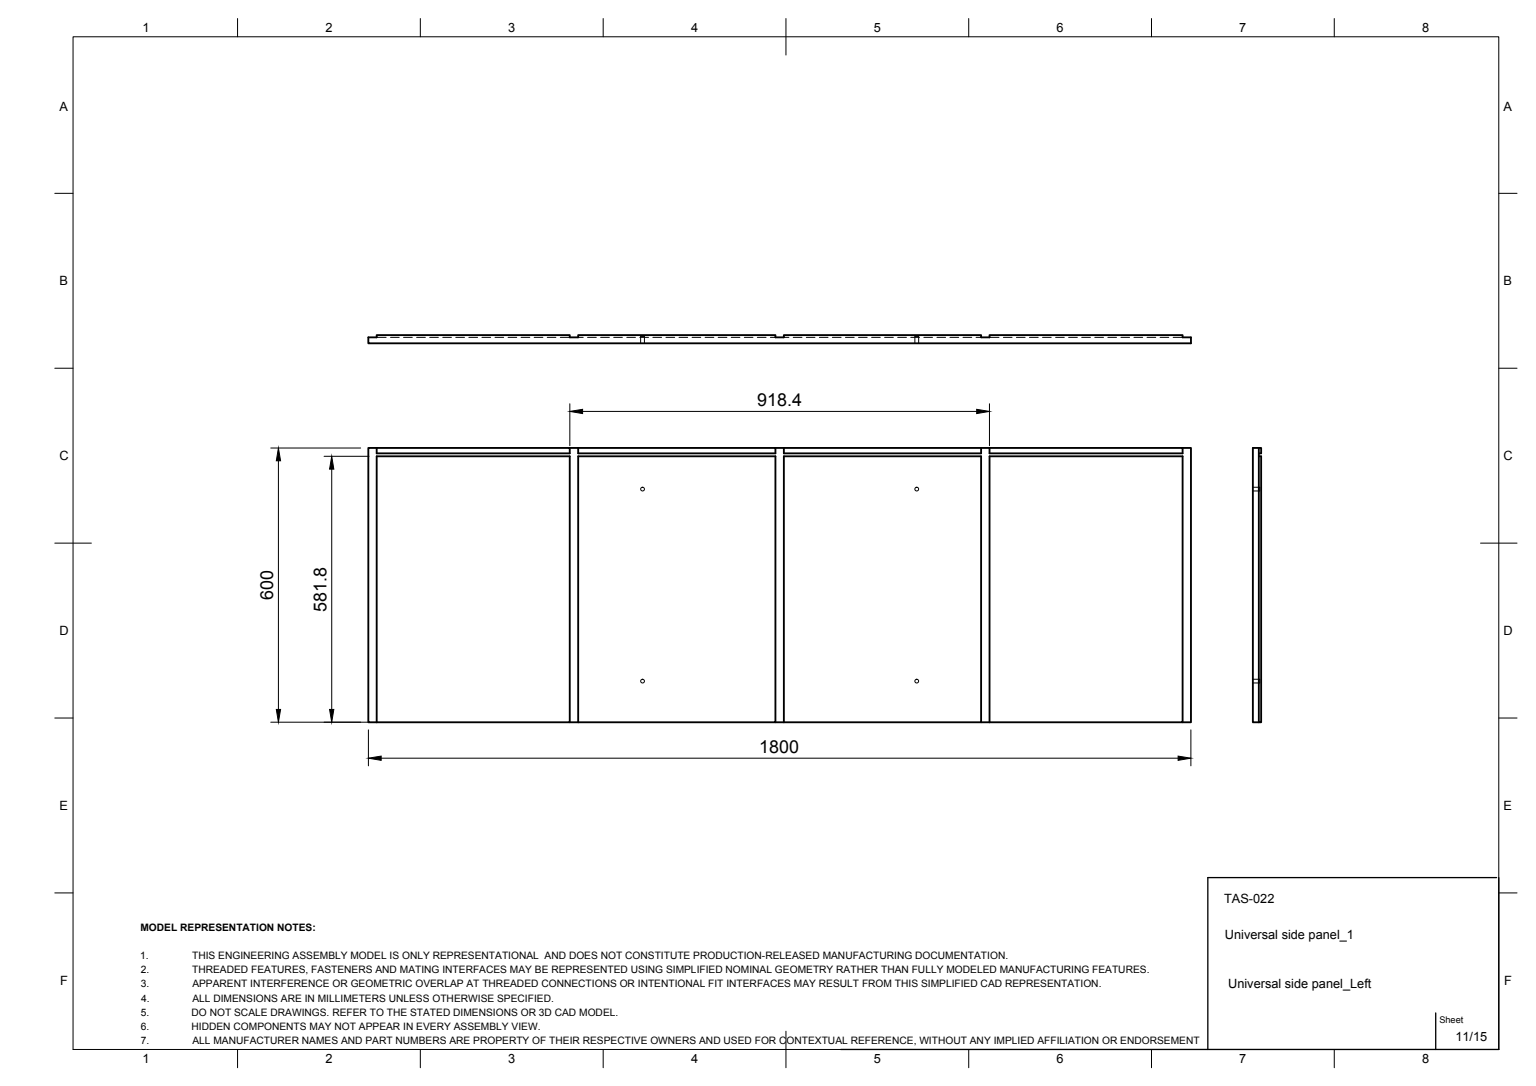
ISO-10303-21;
HEADER;
/* Generated by software containing ST-Developer
 * from STEP Tools, Inc. (www.steptools.com) 
 */

FILE_DESCRIPTION(
/* description */ (''),
/* implementation_level */ '2;1');

FILE_NAME(
/* name */ 'Universal side panel_Left.step',
/* time_stamp */ '2026-11-15T21:02:08-08:00',
/* author */ (''),
/* organization */ (''),
/* preprocessor_version */ 'ST-DEVELOPER v20.2',
/* originating_system */ 'Autodesk Translation Framework v15.17.0.0',
/* authorisation */ '');

FILE_SCHEMA (('AUTOMOTIVE_DESIGN { 1 0 10303 214 3 1 1 }'));
ENDSEC;

DATA;
#10=MECHANICAL_DESIGN_GEOMETRIC_PRESENTATION_REPRESENTATION('',(#613),#31566);
#413=FACE_BOUND('',#1182,.T.);
#414=FACE_BOUND('',#1183,.T.);
#415=FACE_BOUND('',#1184,.T.);
#416=FACE_BOUND('',#1185,.T.);
#480=CIRCLE('',#6173,0.409999999999997);
#481=CIRCLE('',#6174,0.409999999999997);
#482=CIRCLE('',#6177,0.409999999999997);
#483=CIRCLE('',#6178,0.409999999999997);
#484=CIRCLE('',#6181,0.409999999999997);
#485=CIRCLE('',#6182,0.409999999999997);
#486=CIRCLE('',#6185,0.409999999999997);
#487=CIRCLE('',#6186,0.409999999999997);
#567=CYLINDRICAL_SURFACE('',#6172,0.409999999999997);
#568=CYLINDRICAL_SURFACE('',#6176,0.409999999999997);
#569=CYLINDRICAL_SURFACE('',#6180,0.409999999999997);
#570=CYLINDRICAL_SURFACE('',#6184,0.409999999999997);
#583=SHAPE_REPRESENTATION_RELATIONSHIP('SRR','None',#31647,#598);
#598=ADVANCED_BREP_SHAPE_REPRESENTATION('',(#628),#31562);
#613=STYLED_ITEM('',(#31723),#628);
#628=MANIFOLD_SOLID_BREP('Body1',#5726);
#836=FACE_OUTER_BOUND('',#1137,.T.);
#837=FACE_OUTER_BOUND('',#1138,.T.);
#838=FACE_OUTER_BOUND('',#1139,.T.);
#839=FACE_OUTER_BOUND('',#1140,.T.);
#840=FACE_OUTER_BOUND('',#1141,.T.);
#841=FACE_OUTER_BOUND('',#1142,.T.);
#842=FACE_OUTER_BOUND('',#1143,.T.);
#843=FACE_OUTER_BOUND('',#1144,.T.);
#844=FACE_OUTER_BOUND('',#1145,.T.);
#845=FACE_OUTER_BOUND('',#1146,.T.);
#846=FACE_OUTER_BOUND('',#1147,.T.);
#847=FACE_OUTER_BOUND('',#1148,.T.);
#848=FACE_OUTER_BOUND('',#1149,.T.);
#849=FACE_OUTER_BOUND('',#1150,.T.);
#850=FACE_OUTER_BOUND('',#1151,.T.);
#851=FACE_OUTER_BOUND('',#1152,.T.);
#852=FACE_OUTER_BOUND('',#1153,.T.);
#853=FACE_OUTER_BOUND('',#1154,.T.);
#854=FACE_OUTER_BOUND('',#1155,.T.);
#855=FACE_OUTER_BOUND('',#1156,.T.);
#856=FACE_OUTER_BOUND('',#1157,.T.);
#857=FACE_OUTER_BOUND('',#1158,.T.);
#858=FACE_OUTER_BOUND('',#1159,.T.);
#859=FACE_OUTER_BOUND('',#1160,.T.);
#860=FACE_OUTER_BOUND('',#1161,.T.);
#861=FACE_OUTER_BOUND('',#1162,.T.);
#862=FACE_OUTER_BOUND('',#1163,.T.);
#863=FACE_OUTER_BOUND('',#1164,.T.);
#864=FACE_OUTER_BOUND('',#1165,.T.);
#865=FACE_OUTER_BOUND('',#1166,.T.);
#866=FACE_OUTER_BOUND('',#1167,.T.);
#867=FACE_OUTER_BOUND('',#1168,.T.);
#868=FACE_OUTER_BOUND('',#1169,.T.);
#869=FACE_OUTER_BOUND('',#1170,.T.);
#870=FACE_OUTER_BOUND('',#1171,.T.);
#871=FACE_OUTER_BOUND('',#1172,.T.);
#872=FACE_OUTER_BOUND('',#1173,.T.);
#873=FACE_OUTER_BOUND('',#1174,.T.);
#874=FACE_OUTER_BOUND('',#1175,.T.);
#875=FACE_OUTER_BOUND('',#1176,.T.);
#876=FACE_OUTER_BOUND('',#1177,.T.);
#877=FACE_OUTER_BOUND('',#1178,.T.);
#878=FACE_OUTER_BOUND('',#1179,.T.);
#879=FACE_OUTER_BOUND('',#1180,.T.);
#880=FACE_OUTER_BOUND('',#1181,.T.);
#881=FACE_OUTER_BOUND('',#1186,.T.);
#1137=EDGE_LOOP('',(#4945,#4946,#4947,#4948));
#1138=EDGE_LOOP('',(#4949));
#1139=EDGE_LOOP('',(#4950,#4951,#4952,#4953));
#1140=EDGE_LOOP('',(#4954));
#1141=EDGE_LOOP('',(#4955,#4956,#4957,#4958));
#1142=EDGE_LOOP('',(#4959));
#1143=EDGE_LOOP('',(#4960,#4961,#4962,#4963));
#1144=EDGE_LOOP('',(#4964));
#1145=EDGE_LOOP('',(#4965,#4966,#4967,#4968));
#1146=EDGE_LOOP('',(#4969,#4970,#4971,#4972));
#1147=EDGE_LOOP('',(#4973,#4974,#4975,#4976));
#1148=EDGE_LOOP('',(#4977,#4978,#4979,#4980));
#1149=EDGE_LOOP('',(#4981,#4982,#4983,#4984));
#1150=EDGE_LOOP('',(#4985,#4986,#4987,#4988));
#1151=EDGE_LOOP('',(#4989,#4990,#4991,#4992));
#1152=EDGE_LOOP('',(#4993,#4994,#4995,#4996));
#1153=EDGE_LOOP('',(#4997,#4998,#4999,#5000,#5001,#5002,#5003,#5004,#5005,
#5006,#5007,#5008,#5009,#5010,#5011,#5012,#5013,#5014,#5015,#5016,#5017,
#5018,#5019,#5020,#5021,#5022,#5023,#5024,#5025,#5026,#5027,#5028,#5029,
#5030,#5031,#5032));
#1154=EDGE_LOOP('',(#5033,#5034,#5035,#5036));
#1155=EDGE_LOOP('',(#5037,#5038,#5039,#5040));
#1156=EDGE_LOOP('',(#5041,#5042,#5043,#5044));
#1157=EDGE_LOOP('',(#5045,#5046,#5047,#5048));
#1158=EDGE_LOOP('',(#5049,#5050,#5051,#5052));
#1159=EDGE_LOOP('',(#5053,#5054,#5055,#5056));
#1160=EDGE_LOOP('',(#5057,#5058,#5059,#5060));
#1161=EDGE_LOOP('',(#5061,#5062,#5063,#5064));
#1162=EDGE_LOOP('',(#5065,#5066,#5067,#5068));
#1163=EDGE_LOOP('',(#5069,#5070,#5071,#5072));
#1164=EDGE_LOOP('',(#5073,#5074,#5075,#5076));
#1165=EDGE_LOOP('',(#5077,#5078,#5079,#5080));
#1166=EDGE_LOOP('',(#5081,#5082,#5083,#5084));
#1167=EDGE_LOOP('',(#5085,#5086,#5087,#5088));
#1168=EDGE_LOOP('',(#5089,#5090,#5091,#5092));
#1169=EDGE_LOOP('',(#5093,#5094,#5095,#5096));
#1170=EDGE_LOOP('',(#5097,#5098,#5099,#5100));
#1171=EDGE_LOOP('',(#5101,#5102,#5103,#5104));
#1172=EDGE_LOOP('',(#5105,#5106,#5107,#5108));
#1173=EDGE_LOOP('',(#5109,#5110,#5111,#5112));
#1174=EDGE_LOOP('',(#5113,#5114,#5115,#5116));
#1175=EDGE_LOOP('',(#5117,#5118,#5119,#5120));
#1176=EDGE_LOOP('',(#5121,#5122,#5123,#5124));
#1177=EDGE_LOOP('',(#5125,#5126,#5127,#5128));
#1178=EDGE_LOOP('',(#5129,#5130,#5131,#5132,#5133,#5134,#5135,#5136,#5137,
#5138,#5139,#5140,#5141,#5142,#5143,#5144,#5145,#5146,#5147,#5148));
#1179=EDGE_LOOP('',(#5149,#5150,#5151,#5152));
#1180=EDGE_LOOP('',(#5153,#5154,#5155,#5156,#5157,#5158,#5159,#5160,#5161,
#5162,#5163,#5164,#5165,#5166,#5167,#5168,#5169,#5170,#5171,#5172));
#1181=EDGE_LOOP('',(#5173,#5174,#5175,#5176));
#1182=EDGE_LOOP('',(#5177));
#1183=EDGE_LOOP('',(#5178));
#1184=EDGE_LOOP('',(#5179));
#1185=EDGE_LOOP('',(#5180));
#1186=EDGE_LOOP('',(#5181,#5182,#5183,#5184));
#1564=LINE('',#31172,#2071);
#1565=LINE('',#31179,#2072);
#1566=LINE('',#31186,#2073);
#1567=LINE('',#31193,#2074);
#1568=LINE('',#31199,#2075);
#1569=LINE('',#31201,#2076);
#1570=LINE('',#31203,#2077);
#1571=LINE('',#31204,#2078);
#1572=LINE('',#31208,#2079);
#1573=LINE('',#31210,#2080);
#1574=LINE('',#31212,#2081);
#1575=LINE('',#31213,#2082);
#1576=LINE('',#31217,#2083);
#1577=LINE('',#31219,#2084);
#1578=LINE('',#31221,#2085);
#1579=LINE('',#31222,#2086);
#1580=LINE('',#31226,#2087);
#1581=LINE('',#31228,#2088);
#1582=LINE('',#31230,#2089);
#1583=LINE('',#31231,#2090);
#1584=LINE('',#31235,#2091);
#1585=LINE('',#31237,#2092);
#1586=LINE('',#31239,#2093);
#1587=LINE('',#31240,#2094);
#1588=LINE('',#31244,#2095);
#1589=LINE('',#31246,#2096);
#1590=LINE('',#31248,#2097);
#1591=LINE('',#31249,#2098);
#1592=LINE('',#31253,#2099);
#1593=LINE('',#31255,#2100);
#1594=LINE('',#31257,#2101);
#1595=LINE('',#31258,#2102);
#1596=LINE('',#31262,#2103);
#1597=LINE('',#31264,#2104);
#1598=LINE('',#31266,#2105);
#1599=LINE('',#31267,#2106);
#1600=LINE('',#31270,#2107);
#1601=LINE('',#31272,#2108);
#1602=LINE('',#31274,#2109);
#1603=LINE('',#31276,#2110);
#1604=LINE('',#31277,#2111);
#1605=LINE('',#31279,#2112);
#1606=LINE('',#31281,#2113);
#1607=LINE('',#31282,#2114);
#1608=LINE('',#31284,#2115);
#1609=LINE('',#31286,#2116);
#1610=LINE('',#31287,#2117);
#1611=LINE('',#31289,#2118);
#1612=LINE('',#31291,#2119);
#1613=LINE('',#31292,#2120);
#1614=LINE('',#31294,#2121);
#1615=LINE('',#31296,#2122);
#1616=LINE('',#31298,#2123);
#1617=LINE('',#31300,#2124);
#1618=LINE('',#31301,#2125);
#1619=LINE('',#31303,#2126);
#1620=LINE('',#31305,#2127);
#1621=LINE('',#31306,#2128);
#1622=LINE('',#31308,#2129);
#1623=LINE('',#31310,#2130);
#1624=LINE('',#31311,#2131);
#1625=LINE('',#31313,#2132);
#1626=LINE('',#31315,#2133);
#1627=LINE('',#31316,#2134);
#1628=LINE('',#31319,#2135);
#1629=LINE('',#31320,#2136);
#1630=LINE('',#31323,#2137);
#1631=LINE('',#31324,#2138);
#1632=LINE('',#31327,#2139);
#1633=LINE('',#31328,#2140);
#1634=LINE('',#31331,#2141);
#1635=LINE('',#31332,#2142);
#1636=LINE('',#31334,#2143);
#1637=LINE('',#31336,#2144);
#1638=LINE('',#31339,#2145);
#1639=LINE('',#31340,#2146);
#1640=LINE('',#31343,#2147);
#1641=LINE('',#31344,#2148);
#1642=LINE('',#31347,#2149);
#1643=LINE('',#31348,#2150);
#1644=LINE('',#31351,#2151);
#1645=LINE('',#31352,#2152);
#1646=LINE('',#31354,#2153);
#1647=LINE('',#31356,#2154);
#1648=LINE('',#31359,#2155);
#1649=LINE('',#31360,#2156);
#1650=LINE('',#31363,#2157);
#1651=LINE('',#31364,#2158);
#1652=LINE('',#31367,#2159);
#1653=LINE('',#31368,#2160);
#1654=LINE('',#31371,#2161);
#1655=LINE('',#31372,#2162);
#1656=LINE('',#31374,#2163);
#1657=LINE('',#31376,#2164);
#1658=LINE('',#31379,#2165);
#1659=LINE('',#31380,#2166);
#1660=LINE('',#31383,#2167);
#1661=LINE('',#31384,#2168);
#1662=LINE('',#31387,#2169);
#1663=LINE('',#31388,#2170);
#1664=LINE('',#31391,#2171);
#1665=LINE('',#31392,#2172);
#1666=LINE('',#31394,#2173);
#1667=LINE('',#31396,#2174);
#1668=LINE('',#31399,#2175);
#1669=LINE('',#31401,#2176);
#1670=LINE('',#31402,#2177);
#1671=LINE('',#31405,#2178);
#1672=LINE('',#31406,#2179);
#1673=LINE('',#31409,#2180);
#1674=LINE('',#31410,#2181);
#1675=LINE('',#31412,#2182);
#2071=VECTOR('',#7196,0.409999999999997);
#2072=VECTOR('',#7205,0.409999999999997);
#2073=VECTOR('',#7214,0.409999999999997);
#2074=VECTOR('',#7223,0.409999999999997);
#2075=VECTOR('',#7230,1.);
#2076=VECTOR('',#7231,1.);
#2077=VECTOR('',#7232,1.);
#2078=VECTOR('',#7233,1.);
#2079=VECTOR('',#7236,1.);
#2080=VECTOR('',#7237,1.);
#2081=VECTOR('',#7238,1.);
#2082=VECTOR('',#7239,1.);
#2083=VECTOR('',#7242,1.);
#2084=VECTOR('',#7243,1.);
#2085=VECTOR('',#7244,1.);
#2086=VECTOR('',#7245,1.);
#2087=VECTOR('',#7248,1.);
#2088=VECTOR('',#7249,1.);
#2089=VECTOR('',#7250,1.);
#2090=VECTOR('',#7251,1.);
#2091=VECTOR('',#7254,1.);
#2092=VECTOR('',#7255,1.);
#2093=VECTOR('',#7256,1.);
#2094=VECTOR('',#7257,1.);
#2095=VECTOR('',#7260,1.);
#2096=VECTOR('',#7261,1.);
#2097=VECTOR('',#7262,1.);
#2098=VECTOR('',#7263,1.);
#2099=VECTOR('',#7266,1.);
#2100=VECTOR('',#7267,1.);
#2101=VECTOR('',#7268,1.);
#2102=VECTOR('',#7269,1.);
#2103=VECTOR('',#7272,1.);
#2104=VECTOR('',#7273,1.);
#2105=VECTOR('',#7274,1.);
#2106=VECTOR('',#7275,1.);
#2107=VECTOR('',#7278,1.);
#2108=VECTOR('',#7279,1.);
#2109=VECTOR('',#7280,1.);
#2110=VECTOR('',#7281,1.);
#2111=VECTOR('',#7282,1.);
#2112=VECTOR('',#7283,1.);
#2113=VECTOR('',#7284,1.);
#2114=VECTOR('',#7285,1.);
#2115=VECTOR('',#7286,1.);
#2116=VECTOR('',#7287,1.);
#2117=VECTOR('',#7288,1.);
#2118=VECTOR('',#7289,1.);
#2119=VECTOR('',#7290,1.);
#2120=VECTOR('',#7291,1.);
#2121=VECTOR('',#7292,1.);
#2122=VECTOR('',#7293,1.);
#2123=VECTOR('',#7294,1.);
#2124=VECTOR('',#7295,1.);
#2125=VECTOR('',#7296,1.);
#2126=VECTOR('',#7297,1.);
#2127=VECTOR('',#7298,1.);
#2128=VECTOR('',#7299,1.);
#2129=VECTOR('',#7300,1.);
#2130=VECTOR('',#7301,1.);
#2131=VECTOR('',#7302,1.);
#2132=VECTOR('',#7303,1.);
#2133=VECTOR('',#7304,1.);
#2134=VECTOR('',#7305,1.);
#2135=VECTOR('',#7308,1.);
#2136=VECTOR('',#7309,1.);
#2137=VECTOR('',#7312,1.);
#2138=VECTOR('',#7313,1.);
#2139=VECTOR('',#7316,1.);
#2140=VECTOR('',#7317,1.);
#2141=VECTOR('',#7320,1.);
#2142=VECTOR('',#7321,1.);
#2143=VECTOR('',#7324,1.);
#2144=VECTOR('',#7327,1.);
#2145=VECTOR('',#7330,1.);
#2146=VECTOR('',#7331,1.);
#2147=VECTOR('',#7334,1.);
#2148=VECTOR('',#7335,1.);
#2149=VECTOR('',#7338,1.);
#2150=VECTOR('',#7339,1.);
#2151=VECTOR('',#7342,1.);
#2152=VECTOR('',#7343,1.);
#2153=VECTOR('',#7346,1.);
#2154=VECTOR('',#7349,1.);
#2155=VECTOR('',#7352,1.);
#2156=VECTOR('',#7353,1.);
#2157=VECTOR('',#7356,1.);
#2158=VECTOR('',#7357,1.);
#2159=VECTOR('',#7360,1.);
#2160=VECTOR('',#7361,1.);
#2161=VECTOR('',#7364,1.);
#2162=VECTOR('',#7365,1.);
#2163=VECTOR('',#7368,1.);
#2164=VECTOR('',#7371,1.);
#2165=VECTOR('',#7374,1.);
#2166=VECTOR('',#7375,1.);
#2167=VECTOR('',#7378,1.);
#2168=VECTOR('',#7379,1.);
#2169=VECTOR('',#7382,1.);
#2170=VECTOR('',#7383,1.);
#2171=VECTOR('',#7386,1.);
#2172=VECTOR('',#7387,1.);
#2173=VECTOR('',#7390,1.);
#2174=VECTOR('',#7393,1.);
#2175=VECTOR('',#7396,1.);
#2176=VECTOR('',#7397,1.);
#2177=VECTOR('',#7398,1.);
#2178=VECTOR('',#7401,1.);
#2179=VECTOR('',#7402,1.);
#2180=VECTOR('',#7405,1.);
#2181=VECTOR('',#7406,1.);
#2182=VECTOR('',#7409,1.);
#2703=VERTEX_POINT('',#31169);
#2704=VERTEX_POINT('',#31171);
#2705=VERTEX_POINT('',#31176);
#2706=VERTEX_POINT('',#31178);
#2707=VERTEX_POINT('',#31183);
#2708=VERTEX_POINT('',#31185);
#2709=VERTEX_POINT('',#31190);
#2710=VERTEX_POINT('',#31192);
#2711=VERTEX_POINT('',#31197);
#2712=VERTEX_POINT('',#31198);
#2713=VERTEX_POINT('',#31200);
#2714=VERTEX_POINT('',#31202);
#2715=VERTEX_POINT('',#31206);
#2716=VERTEX_POINT('',#31207);
#2717=VERTEX_POINT('',#31209);
#2718=VERTEX_POINT('',#31211);
#2719=VERTEX_POINT('',#31215);
#2720=VERTEX_POINT('',#31216);
#2721=VERTEX_POINT('',#31218);
#2722=VERTEX_POINT('',#31220);
#2723=VERTEX_POINT('',#31224);
#2724=VERTEX_POINT('',#31225);
#2725=VERTEX_POINT('',#31227);
#2726=VERTEX_POINT('',#31229);
#2727=VERTEX_POINT('',#31233);
#2728=VERTEX_POINT('',#31234);
#2729=VERTEX_POINT('',#31236);
#2730=VERTEX_POINT('',#31238);
#2731=VERTEX_POINT('',#31242);
#2732=VERTEX_POINT('',#31243);
#2733=VERTEX_POINT('',#31245);
#2734=VERTEX_POINT('',#31247);
#2735=VERTEX_POINT('',#31251);
#2736=VERTEX_POINT('',#31252);
#2737=VERTEX_POINT('',#31254);
#2738=VERTEX_POINT('',#31256);
#2739=VERTEX_POINT('',#31260);
#2740=VERTEX_POINT('',#31261);
#2741=VERTEX_POINT('',#31263);
#2742=VERTEX_POINT('',#31265);
#2743=VERTEX_POINT('',#31269);
#2744=VERTEX_POINT('',#31271);
#2745=VERTEX_POINT('',#31273);
#2746=VERTEX_POINT('',#31275);
#2747=VERTEX_POINT('',#31278);
#2748=VERTEX_POINT('',#31280);
#2749=VERTEX_POINT('',#31283);
#2750=VERTEX_POINT('',#31285);
#2751=VERTEX_POINT('',#31288);
#2752=VERTEX_POINT('',#31290);
#2753=VERTEX_POINT('',#31293);
#2754=VERTEX_POINT('',#31295);
#2755=VERTEX_POINT('',#31297);
#2756=VERTEX_POINT('',#31299);
#2757=VERTEX_POINT('',#31302);
#2758=VERTEX_POINT('',#31304);
#2759=VERTEX_POINT('',#31307);
#2760=VERTEX_POINT('',#31309);
#2761=VERTEX_POINT('',#31312);
#2762=VERTEX_POINT('',#31314);
#2763=VERTEX_POINT('',#31318);
#2764=VERTEX_POINT('',#31322);
#2765=VERTEX_POINT('',#31326);
#2766=VERTEX_POINT('',#31330);
#2767=VERTEX_POINT('',#31338);
#2768=VERTEX_POINT('',#31342);
#2769=VERTEX_POINT('',#31346);
#2770=VERTEX_POINT('',#31350);
#2771=VERTEX_POINT('',#31358);
#2772=VERTEX_POINT('',#31362);
#2773=VERTEX_POINT('',#31366);
#2774=VERTEX_POINT('',#31370);
#2775=VERTEX_POINT('',#31378);
#2776=VERTEX_POINT('',#31382);
#2777=VERTEX_POINT('',#31386);
#2778=VERTEX_POINT('',#31390);
#2779=VERTEX_POINT('',#31398);
#2780=VERTEX_POINT('',#31400);
#2781=VERTEX_POINT('',#31404);
#2782=VERTEX_POINT('',#31408);
#3468=EDGE_CURVE('',#2703,#2703,#480,.T.);
#3469=EDGE_CURVE('',#2703,#2704,#1564,.T.);
#3470=EDGE_CURVE('',#2704,#2704,#481,.T.);
#3471=EDGE_CURVE('',#2705,#2705,#482,.T.);
#3472=EDGE_CURVE('',#2705,#2706,#1565,.T.);
#3473=EDGE_CURVE('',#2706,#2706,#483,.T.);
#3474=EDGE_CURVE('',#2707,#2707,#484,.T.);
#3475=EDGE_CURVE('',#2707,#2708,#1566,.T.);
#3476=EDGE_CURVE('',#2708,#2708,#485,.T.);
#3477=EDGE_CURVE('',#2709,#2709,#486,.T.);
#3478=EDGE_CURVE('',#2709,#2710,#1567,.T.);
#3479=EDGE_CURVE('',#2710,#2710,#487,.T.);
#3480=EDGE_CURVE('',#2711,#2712,#1568,.T.);
#3481=EDGE_CURVE('',#2713,#2711,#1569,.T.);
#3482=EDGE_CURVE('',#2714,#2713,#1570,.T.);
#3483=EDGE_CURVE('',#2712,#2714,#1571,.T.);
#3484=EDGE_CURVE('',#2715,#2716,#1572,.T.);
#3485=EDGE_CURVE('',#2717,#2715,#1573,.T.);
#3486=EDGE_CURVE('',#2718,#2717,#1574,.T.);
#3487=EDGE_CURVE('',#2716,#2718,#1575,.T.);
#3488=EDGE_CURVE('',#2719,#2720,#1576,.T.);
#3489=EDGE_CURVE('',#2721,#2719,#1577,.T.);
#3490=EDGE_CURVE('',#2722,#2721,#1578,.T.);
#3491=EDGE_CURVE('',#2720,#2722,#1579,.T.);
#3492=EDGE_CURVE('',#2723,#2724,#1580,.T.);
#3493=EDGE_CURVE('',#2725,#2723,#1581,.T.);
#3494=EDGE_CURVE('',#2726,#2725,#1582,.T.);
#3495=EDGE_CURVE('',#2724,#2726,#1583,.T.);
#3496=EDGE_CURVE('',#2727,#2728,#1584,.T.);
#3497=EDGE_CURVE('',#2729,#2727,#1585,.T.);
#3498=EDGE_CURVE('',#2730,#2729,#1586,.T.);
#3499=EDGE_CURVE('',#2730,#2728,#1587,.T.);
#3500=EDGE_CURVE('',#2731,#2732,#1588,.T.);
#3501=EDGE_CURVE('',#2733,#2731,#1589,.T.);
#3502=EDGE_CURVE('',#2734,#2733,#1590,.T.);
#3503=EDGE_CURVE('',#2734,#2732,#1591,.T.);
#3504=EDGE_CURVE('',#2735,#2736,#1592,.T.);
#3505=EDGE_CURVE('',#2737,#2735,#1593,.T.);
#3506=EDGE_CURVE('',#2738,#2737,#1594,.T.);
#3507=EDGE_CURVE('',#2738,#2736,#1595,.T.);
#3508=EDGE_CURVE('',#2739,#2740,#1596,.T.);
#3509=EDGE_CURVE('',#2741,#2739,#1597,.T.);
#3510=EDGE_CURVE('',#2742,#2741,#1598,.T.);
#3511=EDGE_CURVE('',#2742,#2740,#1599,.T.);
#3512=EDGE_CURVE('',#2743,#2723,#1600,.T.);
#3513=EDGE_CURVE('',#2744,#2743,#1601,.T.);
#3514=EDGE_CURVE('',#2745,#2744,#1602,.T.);
#3515=EDGE_CURVE('',#2746,#2745,#1603,.T.);
#3516=EDGE_CURVE('',#2740,#2746,#1604,.T.);
#3517=EDGE_CURVE('',#2742,#2747,#1605,.T.);
#3518=EDGE_CURVE('',#2748,#2747,#1606,.T.);
#3519=EDGE_CURVE('',#2736,#2748,#1607,.T.);
#3520=EDGE_CURVE('',#2738,#2749,#1608,.T.);
#3521=EDGE_CURVE('',#2750,#2749,#1609,.T.);
#3522=EDGE_CURVE('',#2732,#2750,#1610,.T.);
#3523=EDGE_CURVE('',#2734,#2751,#1611,.T.);
#3524=EDGE_CURVE('',#2752,#2751,#1612,.T.);
#3525=EDGE_CURVE('',#2728,#2752,#1613,.T.);
#3526=EDGE_CURVE('',#2730,#2753,#1614,.T.);
#3527=EDGE_CURVE('',#2754,#2753,#1615,.T.);
#3528=EDGE_CURVE('',#2755,#2754,#1616,.T.);
#3529=EDGE_CURVE('',#2756,#2755,#1617,.T.);
#3530=EDGE_CURVE('',#2756,#2721,#1618,.T.);
#3531=EDGE_CURVE('',#2757,#2719,#1619,.T.);
#3532=EDGE_CURVE('',#2758,#2757,#1620,.T.);
#3533=EDGE_CURVE('',#2758,#2717,#1621,.T.);
#3534=EDGE_CURVE('',#2759,#2715,#1622,.T.);
#3535=EDGE_CURVE('',#2760,#2759,#1623,.T.);
#3536=EDGE_CURVE('',#2760,#2713,#1624,.T.);
#3537=EDGE_CURVE('',#2761,#2711,#1625,.T.);
#3538=EDGE_CURVE('',#2762,#2761,#1626,.T.);
#3539=EDGE_CURVE('',#2762,#2725,#1627,.T.);
#3540=EDGE_CURVE('',#2763,#2746,#1628,.T.);
#3541=EDGE_CURVE('',#2739,#2763,#1629,.T.);
#3542=EDGE_CURVE('',#2764,#2724,#1630,.T.);
#3543=EDGE_CURVE('',#2743,#2764,#1631,.T.);
#3544=EDGE_CURVE('',#2765,#2763,#1632,.T.);
#3545=EDGE_CURVE('',#2765,#2741,#1633,.T.);
#3546=EDGE_CURVE('',#2726,#2766,#1634,.T.);
#3547=EDGE_CURVE('',#2766,#2764,#1635,.T.);
#3548=EDGE_CURVE('',#2747,#2765,#1636,.T.);
#3549=EDGE_CURVE('',#2766,#2762,#1637,.T.);
#3550=EDGE_CURVE('',#2767,#2748,#1638,.T.);
#3551=EDGE_CURVE('',#2735,#2767,#1639,.T.);
#3552=EDGE_CURVE('',#2768,#2712,#1640,.T.);
#3553=EDGE_CURVE('',#2761,#2768,#1641,.T.);
#3554=EDGE_CURVE('',#2769,#2767,#1642,.T.);
#3555=EDGE_CURVE('',#2769,#2737,#1643,.T.);
#3556=EDGE_CURVE('',#2714,#2770,#1644,.T.);
#3557=EDGE_CURVE('',#2770,#2768,#1645,.T.);
#3558=EDGE_CURVE('',#2749,#2769,#1646,.T.);
#3559=EDGE_CURVE('',#2770,#2760,#1647,.T.);
#3560=EDGE_CURVE('',#2771,#2750,#1648,.T.);
#3561=EDGE_CURVE('',#2731,#2771,#1649,.T.);
#3562=EDGE_CURVE('',#2772,#2716,#1650,.T.);
#3563=EDGE_CURVE('',#2759,#2772,#1651,.T.);
#3564=EDGE_CURVE('',#2773,#2771,#1652,.T.);
#3565=EDGE_CURVE('',#2773,#2733,#1653,.T.);
#3566=EDGE_CURVE('',#2718,#2774,#1654,.T.);
#3567=EDGE_CURVE('',#2774,#2772,#1655,.T.);
#3568=EDGE_CURVE('',#2751,#2773,#1656,.T.);
#3569=EDGE_CURVE('',#2774,#2758,#1657,.T.);
#3570=EDGE_CURVE('',#2775,#2752,#1658,.T.);
#3571=EDGE_CURVE('',#2727,#2775,#1659,.T.);
#3572=EDGE_CURVE('',#2776,#2720,#1660,.T.);
#3573=EDGE_CURVE('',#2757,#2776,#1661,.T.);
#3574=EDGE_CURVE('',#2777,#2775,#1662,.T.);
#3575=EDGE_CURVE('',#2777,#2729,#1663,.T.);
#3576=EDGE_CURVE('',#2722,#2778,#1664,.T.);
#3577=EDGE_CURVE('',#2778,#2776,#1665,.T.);
#3578=EDGE_CURVE('',#2753,#2777,#1666,.T.);
#3579=EDGE_CURVE('',#2778,#2756,#1667,.T.);
#3580=EDGE_CURVE('',#2755,#2779,#1668,.T.);
#3581=EDGE_CURVE('',#2779,#2780,#1669,.T.);
#3582=EDGE_CURVE('',#2744,#2780,#1670,.T.);
#3583=EDGE_CURVE('',#2781,#2754,#1671,.T.);
#3584=EDGE_CURVE('',#2779,#2781,#1672,.T.);
#3585=EDGE_CURVE('',#2782,#2745,#1673,.T.);
#3586=EDGE_CURVE('',#2781,#2782,#1674,.T.);
#3587=EDGE_CURVE('',#2780,#2782,#1675,.T.);
#4945=ORIENTED_EDGE('',*,*,#3468,.F.);
#4946=ORIENTED_EDGE('',*,*,#3469,.T.);
#4947=ORIENTED_EDGE('',*,*,#3470,.T.);
#4948=ORIENTED_EDGE('',*,*,#3469,.F.);
#4949=ORIENTED_EDGE('',*,*,#3470,.F.);
#4950=ORIENTED_EDGE('',*,*,#3471,.F.);
#4951=ORIENTED_EDGE('',*,*,#3472,.T.);
#4952=ORIENTED_EDGE('',*,*,#3473,.T.);
#4953=ORIENTED_EDGE('',*,*,#3472,.F.);
#4954=ORIENTED_EDGE('',*,*,#3473,.F.);
#4955=ORIENTED_EDGE('',*,*,#3474,.F.);
#4956=ORIENTED_EDGE('',*,*,#3475,.T.);
#4957=ORIENTED_EDGE('',*,*,#3476,.T.);
#4958=ORIENTED_EDGE('',*,*,#3475,.F.);
#4959=ORIENTED_EDGE('',*,*,#3476,.F.);
#4960=ORIENTED_EDGE('',*,*,#3477,.F.);
#4961=ORIENTED_EDGE('',*,*,#3478,.T.);
#4962=ORIENTED_EDGE('',*,*,#3479,.T.);
#4963=ORIENTED_EDGE('',*,*,#3478,.F.);
#4964=ORIENTED_EDGE('',*,*,#3479,.F.);
#4965=ORIENTED_EDGE('',*,*,#3480,.F.);
#4966=ORIENTED_EDGE('',*,*,#3481,.F.);
#4967=ORIENTED_EDGE('',*,*,#3482,.F.);
#4968=ORIENTED_EDGE('',*,*,#3483,.F.);
#4969=ORIENTED_EDGE('',*,*,#3484,.F.);
#4970=ORIENTED_EDGE('',*,*,#3485,.F.);
#4971=ORIENTED_EDGE('',*,*,#3486,.F.);
#4972=ORIENTED_EDGE('',*,*,#3487,.F.);
#4973=ORIENTED_EDGE('',*,*,#3488,.F.);
#4974=ORIENTED_EDGE('',*,*,#3489,.F.);
#4975=ORIENTED_EDGE('',*,*,#3490,.F.);
#4976=ORIENTED_EDGE('',*,*,#3491,.F.);
#4977=ORIENTED_EDGE('',*,*,#3492,.F.);
#4978=ORIENTED_EDGE('',*,*,#3493,.F.);
#4979=ORIENTED_EDGE('',*,*,#3494,.F.);
#4980=ORIENTED_EDGE('',*,*,#3495,.F.);
#4981=ORIENTED_EDGE('',*,*,#3496,.F.);
#4982=ORIENTED_EDGE('',*,*,#3497,.F.);
#4983=ORIENTED_EDGE('',*,*,#3498,.F.);
#4984=ORIENTED_EDGE('',*,*,#3499,.T.);
#4985=ORIENTED_EDGE('',*,*,#3500,.F.);
#4986=ORIENTED_EDGE('',*,*,#3501,.F.);
#4987=ORIENTED_EDGE('',*,*,#3502,.F.);
#4988=ORIENTED_EDGE('',*,*,#3503,.T.);
#4989=ORIENTED_EDGE('',*,*,#3504,.F.);
#4990=ORIENTED_EDGE('',*,*,#3505,.F.);
#4991=ORIENTED_EDGE('',*,*,#3506,.F.);
#4992=ORIENTED_EDGE('',*,*,#3507,.T.);
#4993=ORIENTED_EDGE('',*,*,#3508,.F.);
#4994=ORIENTED_EDGE('',*,*,#3509,.F.);
#4995=ORIENTED_EDGE('',*,*,#3510,.F.);
#4996=ORIENTED_EDGE('',*,*,#3511,.T.);
#4997=ORIENTED_EDGE('',*,*,#3512,.F.);
#4998=ORIENTED_EDGE('',*,*,#3513,.F.);
#4999=ORIENTED_EDGE('',*,*,#3514,.F.);
#5000=ORIENTED_EDGE('',*,*,#3515,.F.);
#5001=ORIENTED_EDGE('',*,*,#3516,.F.);
#5002=ORIENTED_EDGE('',*,*,#3511,.F.);
#5003=ORIENTED_EDGE('',*,*,#3517,.T.);
#5004=ORIENTED_EDGE('',*,*,#3518,.F.);
#5005=ORIENTED_EDGE('',*,*,#3519,.F.);
#5006=ORIENTED_EDGE('',*,*,#3507,.F.);
#5007=ORIENTED_EDGE('',*,*,#3520,.T.);
#5008=ORIENTED_EDGE('',*,*,#3521,.F.);
#5009=ORIENTED_EDGE('',*,*,#3522,.F.);
#5010=ORIENTED_EDGE('',*,*,#3503,.F.);
#5011=ORIENTED_EDGE('',*,*,#3523,.T.);
#5012=ORIENTED_EDGE('',*,*,#3524,.F.);
#5013=ORIENTED_EDGE('',*,*,#3525,.F.);
#5014=ORIENTED_EDGE('',*,*,#3499,.F.);
#5015=ORIENTED_EDGE('',*,*,#3526,.T.);
#5016=ORIENTED_EDGE('',*,*,#3527,.F.);
#5017=ORIENTED_EDGE('',*,*,#3528,.F.);
#5018=ORIENTED_EDGE('',*,*,#3529,.F.);
#5019=ORIENTED_EDGE('',*,*,#3530,.T.);
#5020=ORIENTED_EDGE('',*,*,#3489,.T.);
#5021=ORIENTED_EDGE('',*,*,#3531,.F.);
#5022=ORIENTED_EDGE('',*,*,#3532,.F.);
#5023=ORIENTED_EDGE('',*,*,#3533,.T.);
#5024=ORIENTED_EDGE('',*,*,#3485,.T.);
#5025=ORIENTED_EDGE('',*,*,#3534,.F.);
#5026=ORIENTED_EDGE('',*,*,#3535,.F.);
#5027=ORIENTED_EDGE('',*,*,#3536,.T.);
#5028=ORIENTED_EDGE('',*,*,#3481,.T.);
#5029=ORIENTED_EDGE('',*,*,#3537,.F.);
#5030=ORIENTED_EDGE('',*,*,#3538,.F.);
#5031=ORIENTED_EDGE('',*,*,#3539,.T.);
#5032=ORIENTED_EDGE('',*,*,#3493,.T.);
#5033=ORIENTED_EDGE('',*,*,#3508,.T.);
#5034=ORIENTED_EDGE('',*,*,#3516,.T.);
#5035=ORIENTED_EDGE('',*,*,#3540,.F.);
#5036=ORIENTED_EDGE('',*,*,#3541,.F.);
#5037=ORIENTED_EDGE('',*,*,#3492,.T.);
#5038=ORIENTED_EDGE('',*,*,#3542,.F.);
#5039=ORIENTED_EDGE('',*,*,#3543,.F.);
#5040=ORIENTED_EDGE('',*,*,#3512,.T.);
#5041=ORIENTED_EDGE('',*,*,#3509,.T.);
#5042=ORIENTED_EDGE('',*,*,#3541,.T.);
#5043=ORIENTED_EDGE('',*,*,#3544,.F.);
#5044=ORIENTED_EDGE('',*,*,#3545,.T.);
#5045=ORIENTED_EDGE('',*,*,#3495,.T.);
#5046=ORIENTED_EDGE('',*,*,#3546,.T.);
#5047=ORIENTED_EDGE('',*,*,#3547,.T.);
#5048=ORIENTED_EDGE('',*,*,#3542,.T.);
#5049=ORIENTED_EDGE('',*,*,#3510,.T.);
#5050=ORIENTED_EDGE('',*,*,#3545,.F.);
#5051=ORIENTED_EDGE('',*,*,#3548,.F.);
#5052=ORIENTED_EDGE('',*,*,#3517,.F.);
#5053=ORIENTED_EDGE('',*,*,#3494,.T.);
#5054=ORIENTED_EDGE('',*,*,#3539,.F.);
#5055=ORIENTED_EDGE('',*,*,#3549,.F.);
#5056=ORIENTED_EDGE('',*,*,#3546,.F.);
#5057=ORIENTED_EDGE('',*,*,#3504,.T.);
#5058=ORIENTED_EDGE('',*,*,#3519,.T.);
#5059=ORIENTED_EDGE('',*,*,#3550,.F.);
#5060=ORIENTED_EDGE('',*,*,#3551,.F.);
#5061=ORIENTED_EDGE('',*,*,#3480,.T.);
#5062=ORIENTED_EDGE('',*,*,#3552,.F.);
#5063=ORIENTED_EDGE('',*,*,#3553,.F.);
#5064=ORIENTED_EDGE('',*,*,#3537,.T.);
#5065=ORIENTED_EDGE('',*,*,#3505,.T.);
#5066=ORIENTED_EDGE('',*,*,#3551,.T.);
#5067=ORIENTED_EDGE('',*,*,#3554,.F.);
#5068=ORIENTED_EDGE('',*,*,#3555,.T.);
#5069=ORIENTED_EDGE('',*,*,#3483,.T.);
#5070=ORIENTED_EDGE('',*,*,#3556,.T.);
#5071=ORIENTED_EDGE('',*,*,#3557,.T.);
#5072=ORIENTED_EDGE('',*,*,#3552,.T.);
#5073=ORIENTED_EDGE('',*,*,#3506,.T.);
#5074=ORIENTED_EDGE('',*,*,#3555,.F.);
#5075=ORIENTED_EDGE('',*,*,#3558,.F.);
#5076=ORIENTED_EDGE('',*,*,#3520,.F.);
#5077=ORIENTED_EDGE('',*,*,#3482,.T.);
#5078=ORIENTED_EDGE('',*,*,#3536,.F.);
#5079=ORIENTED_EDGE('',*,*,#3559,.F.);
#5080=ORIENTED_EDGE('',*,*,#3556,.F.);
#5081=ORIENTED_EDGE('',*,*,#3500,.T.);
#5082=ORIENTED_EDGE('',*,*,#3522,.T.);
#5083=ORIENTED_EDGE('',*,*,#3560,.F.);
#5084=ORIENTED_EDGE('',*,*,#3561,.F.);
#5085=ORIENTED_EDGE('',*,*,#3484,.T.);
#5086=ORIENTED_EDGE('',*,*,#3562,.F.);
#5087=ORIENTED_EDGE('',*,*,#3563,.F.);
#5088=ORIENTED_EDGE('',*,*,#3534,.T.);
#5089=ORIENTED_EDGE('',*,*,#3501,.T.);
#5090=ORIENTED_EDGE('',*,*,#3561,.T.);
#5091=ORIENTED_EDGE('',*,*,#3564,.F.);
#5092=ORIENTED_EDGE('',*,*,#3565,.T.);
#5093=ORIENTED_EDGE('',*,*,#3487,.T.);
#5094=ORIENTED_EDGE('',*,*,#3566,.T.);
#5095=ORIENTED_EDGE('',*,*,#3567,.T.);
#5096=ORIENTED_EDGE('',*,*,#3562,.T.);
#5097=ORIENTED_EDGE('',*,*,#3502,.T.);
#5098=ORIENTED_EDGE('',*,*,#3565,.F.);
#5099=ORIENTED_EDGE('',*,*,#3568,.F.);
#5100=ORIENTED_EDGE('',*,*,#3523,.F.);
#5101=ORIENTED_EDGE('',*,*,#3486,.T.);
#5102=ORIENTED_EDGE('',*,*,#3533,.F.);
#5103=ORIENTED_EDGE('',*,*,#3569,.F.);
#5104=ORIENTED_EDGE('',*,*,#3566,.F.);
#5105=ORIENTED_EDGE('',*,*,#3496,.T.);
#5106=ORIENTED_EDGE('',*,*,#3525,.T.);
#5107=ORIENTED_EDGE('',*,*,#3570,.F.);
#5108=ORIENTED_EDGE('',*,*,#3571,.F.);
#5109=ORIENTED_EDGE('',*,*,#3488,.T.);
#5110=ORIENTED_EDGE('',*,*,#3572,.F.);
#5111=ORIENTED_EDGE('',*,*,#3573,.F.);
#5112=ORIENTED_EDGE('',*,*,#3531,.T.);
#5113=ORIENTED_EDGE('',*,*,#3497,.T.);
#5114=ORIENTED_EDGE('',*,*,#3571,.T.);
#5115=ORIENTED_EDGE('',*,*,#3574,.F.);
#5116=ORIENTED_EDGE('',*,*,#3575,.T.);
#5117=ORIENTED_EDGE('',*,*,#3491,.T.);
#5118=ORIENTED_EDGE('',*,*,#3576,.T.);
#5119=ORIENTED_EDGE('',*,*,#3577,.T.);
#5120=ORIENTED_EDGE('',*,*,#3572,.T.);
#5121=ORIENTED_EDGE('',*,*,#3498,.T.);
#5122=ORIENTED_EDGE('',*,*,#3575,.F.);
#5123=ORIENTED_EDGE('',*,*,#3578,.F.);
#5124=ORIENTED_EDGE('',*,*,#3526,.F.);
#5125=ORIENTED_EDGE('',*,*,#3490,.T.);
#5126=ORIENTED_EDGE('',*,*,#3530,.F.);
#5127=ORIENTED_EDGE('',*,*,#3579,.F.);
#5128=ORIENTED_EDGE('',*,*,#3576,.F.);
#5129=ORIENTED_EDGE('',*,*,#3549,.T.);
#5130=ORIENTED_EDGE('',*,*,#3538,.T.);
#5131=ORIENTED_EDGE('',*,*,#3553,.T.);
#5132=ORIENTED_EDGE('',*,*,#3557,.F.);
#5133=ORIENTED_EDGE('',*,*,#3559,.T.);
#5134=ORIENTED_EDGE('',*,*,#3535,.T.);
#5135=ORIENTED_EDGE('',*,*,#3563,.T.);
#5136=ORIENTED_EDGE('',*,*,#3567,.F.);
#5137=ORIENTED_EDGE('',*,*,#3569,.T.);
#5138=ORIENTED_EDGE('',*,*,#3532,.T.);
#5139=ORIENTED_EDGE('',*,*,#3573,.T.);
#5140=ORIENTED_EDGE('',*,*,#3577,.F.);
#5141=ORIENTED_EDGE('',*,*,#3579,.T.);
#5142=ORIENTED_EDGE('',*,*,#3529,.T.);
#5143=ORIENTED_EDGE('',*,*,#3580,.T.);
#5144=ORIENTED_EDGE('',*,*,#3581,.T.);
#5145=ORIENTED_EDGE('',*,*,#3582,.F.);
#5146=ORIENTED_EDGE('',*,*,#3513,.T.);
#5147=ORIENTED_EDGE('',*,*,#3543,.T.);
#5148=ORIENTED_EDGE('',*,*,#3547,.F.);
#5149=ORIENTED_EDGE('',*,*,#3528,.T.);
#5150=ORIENTED_EDGE('',*,*,#3583,.F.);
#5151=ORIENTED_EDGE('',*,*,#3584,.F.);
#5152=ORIENTED_EDGE('',*,*,#3580,.F.);
#5153=ORIENTED_EDGE('',*,*,#3548,.T.);
#5154=ORIENTED_EDGE('',*,*,#3544,.T.);
#5155=ORIENTED_EDGE('',*,*,#3540,.T.);
#5156=ORIENTED_EDGE('',*,*,#3515,.T.);
#5157=ORIENTED_EDGE('',*,*,#3585,.F.);
#5158=ORIENTED_EDGE('',*,*,#3586,.F.);
#5159=ORIENTED_EDGE('',*,*,#3583,.T.);
#5160=ORIENTED_EDGE('',*,*,#3527,.T.);
#5161=ORIENTED_EDGE('',*,*,#3578,.T.);
#5162=ORIENTED_EDGE('',*,*,#3574,.T.);
#5163=ORIENTED_EDGE('',*,*,#3570,.T.);
#5164=ORIENTED_EDGE('',*,*,#3524,.T.);
#5165=ORIENTED_EDGE('',*,*,#3568,.T.);
#5166=ORIENTED_EDGE('',*,*,#3564,.T.);
#5167=ORIENTED_EDGE('',*,*,#3560,.T.);
#5168=ORIENTED_EDGE('',*,*,#3521,.T.);
#5169=ORIENTED_EDGE('',*,*,#3558,.T.);
#5170=ORIENTED_EDGE('',*,*,#3554,.T.);
#5171=ORIENTED_EDGE('',*,*,#3550,.T.);
#5172=ORIENTED_EDGE('',*,*,#3518,.T.);
#5173=ORIENTED_EDGE('',*,*,#3584,.T.);
#5174=ORIENTED_EDGE('',*,*,#3586,.T.);
#5175=ORIENTED_EDGE('',*,*,#3587,.F.);
#5176=ORIENTED_EDGE('',*,*,#3581,.F.);
#5177=ORIENTED_EDGE('',*,*,#3468,.T.);
#5178=ORIENTED_EDGE('',*,*,#3471,.T.);
#5179=ORIENTED_EDGE('',*,*,#3474,.T.);
#5180=ORIENTED_EDGE('',*,*,#3477,.T.);
#5181=ORIENTED_EDGE('',*,*,#3514,.T.);
#5182=ORIENTED_EDGE('',*,*,#3582,.T.);
#5183=ORIENTED_EDGE('',*,*,#3587,.T.);
#5184=ORIENTED_EDGE('',*,*,#3585,.T.);
#5386=PLANE('',#6175);
#5387=PLANE('',#6179);
#5388=PLANE('',#6183);
#5389=PLANE('',#6187);
#5390=PLANE('',#6188);
#5391=PLANE('',#6189);
#5392=PLANE('',#6190);
#5393=PLANE('',#6191);
#5394=PLANE('',#6192);
#5395=PLANE('',#6193);
#5396=PLANE('',#6194);
#5397=PLANE('',#6195);
#5398=PLANE('',#6196);
#5399=PLANE('',#6197);
#5400=PLANE('',#6198);
#5401=PLANE('',#6199);
#5402=PLANE('',#6200);
#5403=PLANE('',#6201);
#5404=PLANE('',#6202);
#5405=PLANE('',#6203);
#5406=PLANE('',#6204);
#5407=PLANE('',#6205);
#5408=PLANE('',#6206);
#5409=PLANE('',#6207);
#5410=PLANE('',#6208);
#5411=PLANE('',#6209);
#5412=PLANE('',#6210);
#5413=PLANE('',#6211);
#5414=PLANE('',#6212);
#5415=PLANE('',#6213);
#5416=PLANE('',#6214);
#5417=PLANE('',#6215);
#5418=PLANE('',#6216);
#5419=PLANE('',#6217);
#5420=PLANE('',#6218);
#5421=PLANE('',#6219);
#5422=PLANE('',#6220);
#5423=PLANE('',#6221);
#5424=PLANE('',#6222);
#5425=PLANE('',#6223);
#5426=PLANE('',#6224);
#5427=PLANE('',#6225);
#5650=ADVANCED_FACE('',(#836),#567,.F.);
#5651=ADVANCED_FACE('',(#837),#5386,.F.);
#5652=ADVANCED_FACE('',(#838),#568,.F.);
#5653=ADVANCED_FACE('',(#839),#5387,.F.);
#5654=ADVANCED_FACE('',(#840),#569,.F.);
#5655=ADVANCED_FACE('',(#841),#5388,.F.);
#5656=ADVANCED_FACE('',(#842),#570,.F.);
#5657=ADVANCED_FACE('',(#843),#5389,.F.);
#5658=ADVANCED_FACE('',(#844),#5390,.F.);
#5659=ADVANCED_FACE('',(#845),#5391,.F.);
#5660=ADVANCED_FACE('',(#846),#5392,.F.);
#5661=ADVANCED_FACE('',(#847),#5393,.F.);
#5662=ADVANCED_FACE('',(#848),#5394,.F.);
#5663=ADVANCED_FACE('',(#849),#5395,.F.);
#5664=ADVANCED_FACE('',(#850),#5396,.F.);
#5665=ADVANCED_FACE('',(#851),#5397,.F.);
#5666=ADVANCED_FACE('',(#852),#5398,.F.);
#5667=ADVANCED_FACE('',(#853),#5399,.T.);
#5668=ADVANCED_FACE('',(#854),#5400,.T.);
#5669=ADVANCED_FACE('',(#855),#5401,.T.);
#5670=ADVANCED_FACE('',(#856),#5402,.T.);
#5671=ADVANCED_FACE('',(#857),#5403,.F.);
#5672=ADVANCED_FACE('',(#858),#5404,.F.);
#5673=ADVANCED_FACE('',(#859),#5405,.T.);
#5674=ADVANCED_FACE('',(#860),#5406,.T.);
#5675=ADVANCED_FACE('',(#861),#5407,.T.);
#5676=ADVANCED_FACE('',(#862),#5408,.T.);
#5677=ADVANCED_FACE('',(#863),#5409,.F.);
#5678=ADVANCED_FACE('',(#864),#5410,.F.);
#5679=ADVANCED_FACE('',(#865),#5411,.T.);
#5680=ADVANCED_FACE('',(#866),#5412,.T.);
#5681=ADVANCED_FACE('',(#867),#5413,.T.);
#5682=ADVANCED_FACE('',(#868),#5414,.T.);
#5683=ADVANCED_FACE('',(#869),#5415,.F.);
#5684=ADVANCED_FACE('',(#870),#5416,.F.);
#5685=ADVANCED_FACE('',(#871),#5417,.T.);
#5686=ADVANCED_FACE('',(#872),#5418,.T.);
#5687=ADVANCED_FACE('',(#873),#5419,.T.);
#5688=ADVANCED_FACE('',(#874),#5420,.T.);
#5689=ADVANCED_FACE('',(#875),#5421,.F.);
#5690=ADVANCED_FACE('',(#876),#5422,.F.);
#5691=ADVANCED_FACE('',(#877),#5423,.T.);
#5692=ADVANCED_FACE('',(#878),#5424,.F.);
#5693=ADVANCED_FACE('',(#879),#5425,.T.);
#5694=ADVANCED_FACE('',(#880,#413,#414,#415,#416),#5426,.T.);
#5695=ADVANCED_FACE('',(#881),#5427,.T.);
#5726=CLOSED_SHELL('',(#5650,#5651,#5652,#5653,#5654,#5655,#5656,#5657,
#5658,#5659,#5660,#5661,#5662,#5663,#5664,#5665,#5666,#5667,#5668,#5669,
#5670,#5671,#5672,#5673,#5674,#5675,#5676,#5677,#5678,#5679,#5680,#5681,
#5682,#5683,#5684,#5685,#5686,#5687,#5688,#5689,#5690,#5691,#5692,#5693,
#5694,#5695));
#6171=AXIS2_PLACEMENT_3D('',#31167,#7190,#7191);
#6172=AXIS2_PLACEMENT_3D('',#31168,#7192,#7193);
#6173=AXIS2_PLACEMENT_3D('',#31170,#7194,#7195);
#6174=AXIS2_PLACEMENT_3D('',#31173,#7197,#7198);
#6175=AXIS2_PLACEMENT_3D('',#31174,#7199,#7200);
#6176=AXIS2_PLACEMENT_3D('',#31175,#7201,#7202);
#6177=AXIS2_PLACEMENT_3D('',#31177,#7203,#7204);
#6178=AXIS2_PLACEMENT_3D('',#31180,#7206,#7207);
#6179=AXIS2_PLACEMENT_3D('',#31181,#7208,#7209);
#6180=AXIS2_PLACEMENT_3D('',#31182,#7210,#7211);
#6181=AXIS2_PLACEMENT_3D('',#31184,#7212,#7213);
#6182=AXIS2_PLACEMENT_3D('',#31187,#7215,#7216);
#6183=AXIS2_PLACEMENT_3D('',#31188,#7217,#7218);
#6184=AXIS2_PLACEMENT_3D('',#31189,#7219,#7220);
#6185=AXIS2_PLACEMENT_3D('',#31191,#7221,#7222);
#6186=AXIS2_PLACEMENT_3D('',#31194,#7224,#7225);
#6187=AXIS2_PLACEMENT_3D('',#31195,#7226,#7227);
#6188=AXIS2_PLACEMENT_3D('',#31196,#7228,#7229);
#6189=AXIS2_PLACEMENT_3D('',#31205,#7234,#7235);
#6190=AXIS2_PLACEMENT_3D('',#31214,#7240,#7241);
#6191=AXIS2_PLACEMENT_3D('',#31223,#7246,#7247);
#6192=AXIS2_PLACEMENT_3D('',#31232,#7252,#7253);
#6193=AXIS2_PLACEMENT_3D('',#31241,#7258,#7259);
#6194=AXIS2_PLACEMENT_3D('',#31250,#7264,#7265);
#6195=AXIS2_PLACEMENT_3D('',#31259,#7270,#7271);
#6196=AXIS2_PLACEMENT_3D('',#31268,#7276,#7277);
#6197=AXIS2_PLACEMENT_3D('',#31317,#7306,#7307);
#6198=AXIS2_PLACEMENT_3D('',#31321,#7310,#7311);
#6199=AXIS2_PLACEMENT_3D('',#31325,#7314,#7315);
#6200=AXIS2_PLACEMENT_3D('',#31329,#7318,#7319);
#6201=AXIS2_PLACEMENT_3D('',#31333,#7322,#7323);
#6202=AXIS2_PLACEMENT_3D('',#31335,#7325,#7326);
#6203=AXIS2_PLACEMENT_3D('',#31337,#7328,#7329);
#6204=AXIS2_PLACEMENT_3D('',#31341,#7332,#7333);
#6205=AXIS2_PLACEMENT_3D('',#31345,#7336,#7337);
#6206=AXIS2_PLACEMENT_3D('',#31349,#7340,#7341);
#6207=AXIS2_PLACEMENT_3D('',#31353,#7344,#7345);
#6208=AXIS2_PLACEMENT_3D('',#31355,#7347,#7348);
#6209=AXIS2_PLACEMENT_3D('',#31357,#7350,#7351);
#6210=AXIS2_PLACEMENT_3D('',#31361,#7354,#7355);
#6211=AXIS2_PLACEMENT_3D('',#31365,#7358,#7359);
#6212=AXIS2_PLACEMENT_3D('',#31369,#7362,#7363);
#6213=AXIS2_PLACEMENT_3D('',#31373,#7366,#7367);
#6214=AXIS2_PLACEMENT_3D('',#31375,#7369,#7370);
#6215=AXIS2_PLACEMENT_3D('',#31377,#7372,#7373);
#6216=AXIS2_PLACEMENT_3D('',#31381,#7376,#7377);
#6217=AXIS2_PLACEMENT_3D('',#31385,#7380,#7381);
#6218=AXIS2_PLACEMENT_3D('',#31389,#7384,#7385);
#6219=AXIS2_PLACEMENT_3D('',#31393,#7388,#7389);
#6220=AXIS2_PLACEMENT_3D('',#31395,#7391,#7392);
#6221=AXIS2_PLACEMENT_3D('',#31397,#7394,#7395);
#6222=AXIS2_PLACEMENT_3D('',#31403,#7399,#7400);
#6223=AXIS2_PLACEMENT_3D('',#31407,#7403,#7404);
#6224=AXIS2_PLACEMENT_3D('',#31411,#7407,#7408);
#6225=AXIS2_PLACEMENT_3D('',#31413,#7410,#7411);
#7190=DIRECTION('axis',(0.,0.,1.));
#7191=DIRECTION('refdir',(1.,0.,0.));
#7192=DIRECTION('center_axis',(1.,0.,0.));
#7193=DIRECTION('ref_axis',(0.,0.,-1.));
#7194=DIRECTION('center_axis',(1.,0.,0.));
#7195=DIRECTION('ref_axis',(0.,0.,-1.));
#7196=DIRECTION('',(1.,0.,0.));
#7197=DIRECTION('center_axis',(1.,0.,0.));
#7198=DIRECTION('ref_axis',(0.,0.,-1.));
#7199=DIRECTION('center_axis',(1.,0.,0.));
#7200=DIRECTION('ref_axis',(0.,0.,-1.));
#7201=DIRECTION('center_axis',(1.,0.,0.));
#7202=DIRECTION('ref_axis',(0.,0.,-1.));
#7203=DIRECTION('center_axis',(1.,0.,0.));
#7204=DIRECTION('ref_axis',(0.,0.,-1.));
#7205=DIRECTION('',(1.,0.,0.));
#7206=DIRECTION('center_axis',(1.,0.,0.));
#7207=DIRECTION('ref_axis',(0.,0.,-1.));
#7208=DIRECTION('center_axis',(1.,0.,0.));
#7209=DIRECTION('ref_axis',(0.,0.,-1.));
#7210=DIRECTION('center_axis',(1.,0.,0.));
#7211=DIRECTION('ref_axis',(0.,0.,-1.));
#7212=DIRECTION('center_axis',(1.,0.,0.));
#7213=DIRECTION('ref_axis',(0.,0.,-1.));
#7214=DIRECTION('',(1.,0.,0.));
#7215=DIRECTION('center_axis',(1.,0.,0.));
#7216=DIRECTION('ref_axis',(0.,0.,-1.));
#7217=DIRECTION('center_axis',(1.,0.,0.));
#7218=DIRECTION('ref_axis',(0.,0.,-1.));
#7219=DIRECTION('center_axis',(1.,0.,0.));
#7220=DIRECTION('ref_axis',(0.,0.,-1.));
#7221=DIRECTION('center_axis',(1.,0.,0.));
#7222=DIRECTION('ref_axis',(0.,0.,-1.));
#7223=DIRECTION('',(1.,0.,0.));
#7224=DIRECTION('center_axis',(1.,0.,0.));
#7225=DIRECTION('ref_axis',(0.,0.,-1.));
#7226=DIRECTION('center_axis',(1.,0.,0.));
#7227=DIRECTION('ref_axis',(0.,0.,-1.));
#7228=DIRECTION('center_axis',(0.,1.,0.));
#7229=DIRECTION('ref_axis',(-1.,0.,0.));
#7230=DIRECTION('',(1.,0.,0.));
#7231=DIRECTION('',(0.,0.,1.));
#7232=DIRECTION('',(-1.,0.,0.));
#7233=DIRECTION('',(0.,0.,-1.));
#7234=DIRECTION('center_axis',(0.,1.,0.));
#7235=DIRECTION('ref_axis',(-1.,0.,0.));
#7236=DIRECTION('',(1.,0.,0.));
#7237=DIRECTION('',(0.,0.,1.));
#7238=DIRECTION('',(-1.,0.,0.));
#7239=DIRECTION('',(0.,0.,-1.));
#7240=DIRECTION('center_axis',(0.,1.,0.));
#7241=DIRECTION('ref_axis',(-1.,0.,0.));
#7242=DIRECTION('',(1.,0.,0.));
#7243=DIRECTION('',(0.,0.,1.));
#7244=DIRECTION('',(-1.,0.,0.));
#7245=DIRECTION('',(0.,0.,-1.));
#7246=DIRECTION('center_axis',(0.,1.,0.));
#7247=DIRECTION('ref_axis',(-1.,0.,0.));
#7248=DIRECTION('',(1.,0.,0.));
#7249=DIRECTION('',(0.,0.,1.));
#7250=DIRECTION('',(-1.,0.,0.));
#7251=DIRECTION('',(0.,0.,-1.));
#7252=DIRECTION('center_axis',(0.,-1.,0.));
#7253=DIRECTION('ref_axis',(1.,0.,0.));
#7254=DIRECTION('',(-1.,0.,0.));
#7255=DIRECTION('',(0.,0.,1.));
#7256=DIRECTION('',(1.,0.,0.));
#7257=DIRECTION('',(0.,0.,1.));
#7258=DIRECTION('center_axis',(0.,-1.,0.));
#7259=DIRECTION('ref_axis',(1.,0.,0.));
#7260=DIRECTION('',(-1.,0.,0.));
#7261=DIRECTION('',(0.,0.,1.));
#7262=DIRECTION('',(1.,0.,0.));
#7263=DIRECTION('',(0.,0.,1.));
#7264=DIRECTION('center_axis',(0.,-1.,0.));
#7265=DIRECTION('ref_axis',(1.,0.,0.));
#7266=DIRECTION('',(-1.,0.,0.));
#7267=DIRECTION('',(0.,0.,1.));
#7268=DIRECTION('',(1.,0.,0.));
#7269=DIRECTION('',(0.,0.,1.));
#7270=DIRECTION('center_axis',(0.,-1.,0.));
#7271=DIRECTION('ref_axis',(1.,0.,0.));
#7272=DIRECTION('',(-1.,0.,0.));
#7273=DIRECTION('',(0.,0.,1.));
#7274=DIRECTION('',(1.,0.,0.));
#7275=DIRECTION('',(0.,0.,1.));
#7276=DIRECTION('center_axis',(-1.,0.,0.));
#7277=DIRECTION('ref_axis',(0.,-1.,0.));
#7278=DIRECTION('',(0.,-1.,0.));
#7279=DIRECTION('',(0.,0.,-1.));
#7280=DIRECTION('',(0.,1.,0.));
#7281=DIRECTION('',(0.,0.,1.));
#7282=DIRECTION('',(0.,-1.,0.));
#7283=DIRECTION('',(0.,-1.,0.));
#7284=DIRECTION('',(0.,0.,1.));
#7285=DIRECTION('',(0.,-1.,0.));
#7286=DIRECTION('',(0.,-1.,0.));
#7287=DIRECTION('',(0.,0.,1.));
#7288=DIRECTION('',(0.,-1.,0.));
#7289=DIRECTION('',(0.,-1.,0.));
#7290=DIRECTION('',(0.,0.,1.));
#7291=DIRECTION('',(0.,-1.,0.));
#7292=DIRECTION('',(0.,-1.,0.));
#7293=DIRECTION('',(0.,0.,1.));
#7294=DIRECTION('',(0.,-1.,0.));
#7295=DIRECTION('',(0.,0.,-1.));
#7296=DIRECTION('',(0.,-1.,0.));
#7297=DIRECTION('',(0.,-1.,0.));
#7298=DIRECTION('',(0.,0.,-1.));
#7299=DIRECTION('',(0.,-1.,0.));
#7300=DIRECTION('',(0.,-1.,0.));
#7301=DIRECTION('',(0.,0.,-1.));
#7302=DIRECTION('',(0.,-1.,0.));
#7303=DIRECTION('',(0.,-1.,0.));
#7304=DIRECTION('',(0.,0.,-1.));
#7305=DIRECTION('',(0.,-1.,0.));
#7306=DIRECTION('center_axis',(0.,0.,1.));
#7307=DIRECTION('ref_axis',(1.,0.,0.));
#7308=DIRECTION('',(-1.,0.,0.));
#7309=DIRECTION('',(0.,-1.,0.));
#7310=DIRECTION('center_axis',(0.,0.,1.));
#7311=DIRECTION('ref_axis',(1.,0.,0.));
#7312=DIRECTION('',(0.,-1.,0.));
#7313=DIRECTION('',(1.,0.,0.));
#7314=DIRECTION('center_axis',(1.,0.,0.));
#7315=DIRECTION('ref_axis',(0.,1.,0.));
#7316=DIRECTION('',(0.,0.,1.));
#7317=DIRECTION('',(0.,1.,0.));
#7318=DIRECTION('center_axis',(1.,0.,0.));
#7319=DIRECTION('ref_axis',(0.,1.,0.));
#7320=DIRECTION('',(0.,1.,0.));
#7321=DIRECTION('',(0.,0.,1.));
#7322=DIRECTION('center_axis',(0.,0.,1.));
#7323=DIRECTION('ref_axis',(1.,0.,0.));
#7324=DIRECTION('',(1.,0.,0.));
#7325=DIRECTION('center_axis',(0.,0.,1.));
#7326=DIRECTION('ref_axis',(1.,0.,0.));
#7327=DIRECTION('',(-1.,0.,0.));
#7328=DIRECTION('center_axis',(0.,0.,1.));
#7329=DIRECTION('ref_axis',(1.,0.,0.));
#7330=DIRECTION('',(-1.,0.,0.));
#7331=DIRECTION('',(0.,-1.,0.));
#7332=DIRECTION('center_axis',(0.,0.,1.));
#7333=DIRECTION('ref_axis',(1.,0.,0.));
#7334=DIRECTION('',(0.,-1.,0.));
#7335=DIRECTION('',(1.,0.,0.));
#7336=DIRECTION('center_axis',(1.,0.,0.));
#7337=DIRECTION('ref_axis',(0.,1.,0.));
#7338=DIRECTION('',(0.,0.,1.));
#7339=DIRECTION('',(0.,1.,0.));
#7340=DIRECTION('center_axis',(1.,0.,0.));
#7341=DIRECTION('ref_axis',(0.,1.,0.));
#7342=DIRECTION('',(0.,1.,0.));
#7343=DIRECTION('',(0.,0.,1.));
#7344=DIRECTION('center_axis',(0.,0.,1.));
#7345=DIRECTION('ref_axis',(1.,0.,0.));
#7346=DIRECTION('',(1.,0.,0.));
#7347=DIRECTION('center_axis',(0.,0.,1.));
#7348=DIRECTION('ref_axis',(1.,0.,0.));
#7349=DIRECTION('',(-1.,0.,0.));
#7350=DIRECTION('center_axis',(0.,0.,1.));
#7351=DIRECTION('ref_axis',(1.,0.,0.));
#7352=DIRECTION('',(-1.,0.,0.));
#7353=DIRECTION('',(0.,-1.,0.));
#7354=DIRECTION('center_axis',(0.,0.,1.));
#7355=DIRECTION('ref_axis',(1.,0.,0.));
#7356=DIRECTION('',(0.,-1.,0.));
#7357=DIRECTION('',(1.,0.,0.));
#7358=DIRECTION('center_axis',(1.,0.,0.));
#7359=DIRECTION('ref_axis',(0.,1.,0.));
#7360=DIRECTION('',(0.,0.,1.));
#7361=DIRECTION('',(0.,1.,0.));
#7362=DIRECTION('center_axis',(1.,0.,0.));
#7363=DIRECTION('ref_axis',(0.,1.,0.));
#7364=DIRECTION('',(0.,1.,0.));
#7365=DIRECTION('',(0.,0.,1.));
#7366=DIRECTION('center_axis',(0.,0.,1.));
#7367=DIRECTION('ref_axis',(1.,0.,0.));
#7368=DIRECTION('',(1.,0.,0.));
#7369=DIRECTION('center_axis',(0.,0.,1.));
#7370=DIRECTION('ref_axis',(1.,0.,0.));
#7371=DIRECTION('',(-1.,0.,0.));
#7372=DIRECTION('center_axis',(0.,0.,1.));
#7373=DIRECTION('ref_axis',(1.,0.,0.));
#7374=DIRECTION('',(-1.,0.,0.));
#7375=DIRECTION('',(0.,-1.,0.));
#7376=DIRECTION('center_axis',(0.,0.,1.));
#7377=DIRECTION('ref_axis',(1.,0.,0.));
#7378=DIRECTION('',(0.,-1.,0.));
#7379=DIRECTION('',(1.,0.,0.));
#7380=DIRECTION('center_axis',(1.,0.,0.));
#7381=DIRECTION('ref_axis',(0.,1.,0.));
#7382=DIRECTION('',(0.,0.,1.));
#7383=DIRECTION('',(0.,1.,0.));
#7384=DIRECTION('center_axis',(1.,0.,0.));
#7385=DIRECTION('ref_axis',(0.,1.,0.));
#7386=DIRECTION('',(0.,1.,0.));
#7387=DIRECTION('',(0.,0.,1.));
#7388=DIRECTION('center_axis',(0.,0.,1.));
#7389=DIRECTION('ref_axis',(1.,0.,0.));
#7390=DIRECTION('',(1.,0.,0.));
#7391=DIRECTION('center_axis',(0.,0.,1.));
#7392=DIRECTION('ref_axis',(1.,0.,0.));
#7393=DIRECTION('',(-1.,0.,0.));
#7394=DIRECTION('center_axis',(0.,1.,0.));
#7395=DIRECTION('ref_axis',(-1.,0.,0.));
#7396=DIRECTION('',(-1.,0.,0.));
#7397=DIRECTION('',(0.,0.,1.));
#7398=DIRECTION('',(-1.,0.,0.));
#7399=DIRECTION('center_axis',(0.,0.,1.));
#7400=DIRECTION('ref_axis',(1.,0.,0.));
#7401=DIRECTION('',(1.,0.,0.));
#7402=DIRECTION('',(0.,-1.,0.));
#7403=DIRECTION('center_axis',(0.,-1.,0.));
#7404=DIRECTION('ref_axis',(1.,0.,0.));
#7405=DIRECTION('',(1.,0.,0.));
#7406=DIRECTION('',(0.,0.,1.));
#7407=DIRECTION('center_axis',(-1.,0.,0.));
#7408=DIRECTION('ref_axis',(0.,-1.,0.));
#7409=DIRECTION('',(0.,-1.,0.));
#7410=DIRECTION('center_axis',(0.,0.,1.));
#7411=DIRECTION('ref_axis',(1.,0.,0.));
#31167=CARTESIAN_POINT('',(0.,0.,0.));
#31168=CARTESIAN_POINT('Origin',(0.,51.,60.));
#31169=CARTESIAN_POINT('',(0.,51.,60.41));
#31170=CARTESIAN_POINT('Origin',(0.,51.,60.));
#31171=CARTESIAN_POINT('',(1.5,51.,60.41));
#31172=CARTESIAN_POINT('',(0.,51.,60.41));
#31173=CARTESIAN_POINT('Origin',(1.5,51.,60.));
#31174=CARTESIAN_POINT('Origin',(1.5,51.,60.));
#31175=CARTESIAN_POINT('Origin',(0.,9.,120.));
#31176=CARTESIAN_POINT('',(0.,9.,120.41));
#31177=CARTESIAN_POINT('Origin',(0.,9.,120.));
#31178=CARTESIAN_POINT('',(1.5,9.,120.41));
#31179=CARTESIAN_POINT('',(0.,9.,120.41));
#31180=CARTESIAN_POINT('Origin',(1.5,9.,120.));
#31181=CARTESIAN_POINT('Origin',(1.5,9.,120.));
#31182=CARTESIAN_POINT('Origin',(0.,9.,60.));
#31183=CARTESIAN_POINT('',(0.,9.,60.41));
#31184=CARTESIAN_POINT('Origin',(0.,9.,60.));
#31185=CARTESIAN_POINT('',(1.5,9.,60.41));
#31186=CARTESIAN_POINT('',(0.,9.,60.41));
#31187=CARTESIAN_POINT('Origin',(1.5,9.,60.));
#31188=CARTESIAN_POINT('Origin',(1.5,9.,60.));
#31189=CARTESIAN_POINT('Origin',(0.,51.,120.));
#31190=CARTESIAN_POINT('',(0.,51.,120.41));
#31191=CARTESIAN_POINT('Origin',(0.,51.,120.));
#31192=CARTESIAN_POINT('',(1.5,51.,120.41));
#31193=CARTESIAN_POINT('',(0.,51.,120.41));
#31194=CARTESIAN_POINT('Origin',(1.5,51.,120.));
#31195=CARTESIAN_POINT('Origin',(1.5,51.,120.));
#31196=CARTESIAN_POINT('Origin',(1.81,58.82,0.));
#31197=CARTESIAN_POINT('',(1.3,58.82,134.08));
#31198=CARTESIAN_POINT('',(1.8,58.82,134.08));
#31199=CARTESIAN_POINT('',(1.6825,58.82,134.08));
#31200=CARTESIAN_POINT('',(1.3,58.82,90.92));
#31201=CARTESIAN_POINT('',(1.3,58.82,0.));
#31202=CARTESIAN_POINT('',(1.8,58.82,90.92));
#31203=CARTESIAN_POINT('',(1.6825,58.82,90.92));
#31204=CARTESIAN_POINT('',(1.8,58.82,0.));
#31205=CARTESIAN_POINT('Origin',(1.81,58.82,0.));
#31206=CARTESIAN_POINT('',(1.3,58.82,89.08));
#31207=CARTESIAN_POINT('',(1.8,58.82,89.08));
#31208=CARTESIAN_POINT('',(1.6825,58.82,89.08));
#31209=CARTESIAN_POINT('',(1.3,58.82,45.92));
#31210=CARTESIAN_POINT('',(1.3,58.82,0.));
#31211=CARTESIAN_POINT('',(1.8,58.82,45.92));
#31212=CARTESIAN_POINT('',(1.6825,58.82,45.92));
#31213=CARTESIAN_POINT('',(1.8,58.82,0.));
#31214=CARTESIAN_POINT('Origin',(1.81,58.82,0.));
#31215=CARTESIAN_POINT('',(1.3,58.82,44.08));
#31216=CARTESIAN_POINT('',(1.8,58.82,44.08));
#31217=CARTESIAN_POINT('',(1.6825,58.82,44.08));
#31218=CARTESIAN_POINT('',(1.3,58.82,1.82));
#31219=CARTESIAN_POINT('',(1.3,58.82,0.));
#31220=CARTESIAN_POINT('',(1.8,58.82,1.82));
#31221=CARTESIAN_POINT('',(1.6825,58.82,1.82));
#31222=CARTESIAN_POINT('',(1.8,58.82,0.));
#31223=CARTESIAN_POINT('Origin',(1.81,58.82,0.));
#31224=CARTESIAN_POINT('',(1.3,58.82,178.18));
#31225=CARTESIAN_POINT('',(1.8,58.82,178.18));
#31226=CARTESIAN_POINT('',(1.6825,58.82,178.18));
#31227=CARTESIAN_POINT('',(1.3,58.82,135.92));
#31228=CARTESIAN_POINT('',(1.3,58.82,0.));
#31229=CARTESIAN_POINT('',(1.8,58.82,135.92));
#31230=CARTESIAN_POINT('',(1.6825,58.82,135.92));
#31231=CARTESIAN_POINT('',(1.8,58.82,0.));
#31232=CARTESIAN_POINT('Origin',(1.3,58.18,0.));
#31233=CARTESIAN_POINT('',(1.8,58.18,44.08));
#31234=CARTESIAN_POINT('',(1.3,58.18,44.08));
#31235=CARTESIAN_POINT('',(1.4275,58.18,44.08));
#31236=CARTESIAN_POINT('',(1.8,58.18,1.82));
#31237=CARTESIAN_POINT('',(1.8,58.18,0.));
#31238=CARTESIAN_POINT('',(1.3,58.18,1.82));
#31239=CARTESIAN_POINT('',(1.4275,58.18,1.82));
#31240=CARTESIAN_POINT('',(1.3,58.18,0.));
#31241=CARTESIAN_POINT('Origin',(1.3,58.18,0.));
#31242=CARTESIAN_POINT('',(1.8,58.18,89.08));
#31243=CARTESIAN_POINT('',(1.3,58.18,89.08));
#31244=CARTESIAN_POINT('',(1.4275,58.18,89.08));
#31245=CARTESIAN_POINT('',(1.8,58.18,45.92));
#31246=CARTESIAN_POINT('',(1.8,58.18,0.));
#31247=CARTESIAN_POINT('',(1.3,58.18,45.92));
#31248=CARTESIAN_POINT('',(1.4275,58.18,45.92));
#31249=CARTESIAN_POINT('',(1.3,58.18,0.));
#31250=CARTESIAN_POINT('Origin',(1.3,58.18,0.));
#31251=CARTESIAN_POINT('',(1.8,58.18,134.08));
#31252=CARTESIAN_POINT('',(1.3,58.18,134.08));
#31253=CARTESIAN_POINT('',(1.4275,58.18,134.08));
#31254=CARTESIAN_POINT('',(1.8,58.18,90.92));
#31255=CARTESIAN_POINT('',(1.8,58.18,0.));
#31256=CARTESIAN_POINT('',(1.3,58.18,90.92));
#31257=CARTESIAN_POINT('',(1.4275,58.18,90.92));
#31258=CARTESIAN_POINT('',(1.3,58.18,0.));
#31259=CARTESIAN_POINT('Origin',(1.3,58.18,0.));
#31260=CARTESIAN_POINT('',(1.8,58.18,178.18));
#31261=CARTESIAN_POINT('',(1.3,58.18,178.18));
#31262=CARTESIAN_POINT('',(1.4275,58.18,178.18));
#31263=CARTESIAN_POINT('',(1.8,58.18,135.92));
#31264=CARTESIAN_POINT('',(1.8,58.18,0.));
#31265=CARTESIAN_POINT('',(1.3,58.18,135.92));
#31266=CARTESIAN_POINT('',(1.4275,58.18,135.92));
#31267=CARTESIAN_POINT('',(1.3,58.18,0.));
#31268=CARTESIAN_POINT('Origin',(1.3,60.,178.18));
#31269=CARTESIAN_POINT('',(1.3,60.,178.18));
#31270=CARTESIAN_POINT('',(1.3,60.,178.18));
#31271=CARTESIAN_POINT('',(1.3,60.,180.));
#31272=CARTESIAN_POINT('',(1.3,60.,89.09));
#31273=CARTESIAN_POINT('',(1.3,0.,180.));
#31274=CARTESIAN_POINT('',(1.3,45.,180.));
#31275=CARTESIAN_POINT('',(1.3,0.,178.18));
#31276=CARTESIAN_POINT('',(1.3,0.,89.09));
#31277=CARTESIAN_POINT('',(1.3,60.,178.18));
#31278=CARTESIAN_POINT('',(1.3,0.,135.92));
#31279=CARTESIAN_POINT('',(1.3,60.,135.92));
#31280=CARTESIAN_POINT('',(1.3,0.,134.08));
#31281=CARTESIAN_POINT('',(1.3,0.,67.04));
#31282=CARTESIAN_POINT('',(1.3,60.,134.08));
#31283=CARTESIAN_POINT('',(1.3,0.,90.92));
#31284=CARTESIAN_POINT('',(1.3,60.,90.92));
#31285=CARTESIAN_POINT('',(1.3,0.,89.08));
#31286=CARTESIAN_POINT('',(1.3,0.,44.54));
#31287=CARTESIAN_POINT('',(1.3,60.,89.08));
#31288=CARTESIAN_POINT('',(1.3,0.,45.92));
#31289=CARTESIAN_POINT('',(1.3,60.,45.92));
#31290=CARTESIAN_POINT('',(1.3,0.,44.08));
#31291=CARTESIAN_POINT('',(1.3,0.,22.04));
#31292=CARTESIAN_POINT('',(1.3,60.,44.08));
#31293=CARTESIAN_POINT('',(1.3,0.,1.82));
#31294=CARTESIAN_POINT('',(1.3,60.,1.82));
#31295=CARTESIAN_POINT('',(1.3,0.,0.));
#31296=CARTESIAN_POINT('',(1.3,0.,0.));
#31297=CARTESIAN_POINT('',(1.3,60.,0.));
#31298=CARTESIAN_POINT('',(1.3,45.,0.));
#31299=CARTESIAN_POINT('',(1.3,60.,1.82));
#31300=CARTESIAN_POINT('',(1.3,60.,0.));
#31301=CARTESIAN_POINT('',(1.3,60.,1.82));
#31302=CARTESIAN_POINT('',(1.3,60.,44.08));
#31303=CARTESIAN_POINT('',(1.3,60.,44.08));
#31304=CARTESIAN_POINT('',(1.3,60.,45.92));
#31305=CARTESIAN_POINT('',(1.3,60.,22.04));
#31306=CARTESIAN_POINT('',(1.3,60.,45.92));
#31307=CARTESIAN_POINT('',(1.3,60.,89.08));
#31308=CARTESIAN_POINT('',(1.3,60.,89.08));
#31309=CARTESIAN_POINT('',(1.3,60.,90.92));
#31310=CARTESIAN_POINT('',(1.3,60.,44.54));
#31311=CARTESIAN_POINT('',(1.3,60.,90.92));
#31312=CARTESIAN_POINT('',(1.3,60.,134.08));
#31313=CARTESIAN_POINT('',(1.3,60.,134.08));
#31314=CARTESIAN_POINT('',(1.3,60.,135.92));
#31315=CARTESIAN_POINT('',(1.3,60.,67.04));
#31316=CARTESIAN_POINT('',(1.3,60.,135.92));
#31317=CARTESIAN_POINT('Origin',(1.555,30.,178.18));
#31318=CARTESIAN_POINT('',(1.8,0.,178.18));
#31319=CARTESIAN_POINT('',(0.7775,0.,178.18));
#31320=CARTESIAN_POINT('',(1.8,15.,178.18));
#31321=CARTESIAN_POINT('Origin',(1.555,30.,178.18));
#31322=CARTESIAN_POINT('',(1.8,60.,178.18));
#31323=CARTESIAN_POINT('',(1.8,15.,178.18));
#31324=CARTESIAN_POINT('',(1.6775,60.,178.18));
#31325=CARTESIAN_POINT('Origin',(1.8,0.,0.));
#31326=CARTESIAN_POINT('',(1.8,0.,135.92));
#31327=CARTESIAN_POINT('',(1.8,0.,0.));
#31328=CARTESIAN_POINT('',(1.8,15.,135.92));
#31329=CARTESIAN_POINT('Origin',(1.8,0.,0.));
#31330=CARTESIAN_POINT('',(1.8,60.,135.92));
#31331=CARTESIAN_POINT('',(1.8,15.,135.92));
#31332=CARTESIAN_POINT('',(1.8,60.,0.));
#31333=CARTESIAN_POINT('Origin',(1.555,30.,135.92));
#31334=CARTESIAN_POINT('',(0.7775,0.,135.92));
#31335=CARTESIAN_POINT('Origin',(1.555,30.,135.92));
#31336=CARTESIAN_POINT('',(1.6775,60.,135.92));
#31337=CARTESIAN_POINT('Origin',(1.555,30.,134.08));
#31338=CARTESIAN_POINT('',(1.8,0.,134.08));
#31339=CARTESIAN_POINT('',(0.7775,0.,134.08));
#31340=CARTESIAN_POINT('',(1.8,15.,134.08));
#31341=CARTESIAN_POINT('Origin',(1.555,30.,134.08));
#31342=CARTESIAN_POINT('',(1.8,60.,134.08));
#31343=CARTESIAN_POINT('',(1.8,15.,134.08));
#31344=CARTESIAN_POINT('',(1.6775,60.,134.08));
#31345=CARTESIAN_POINT('Origin',(1.8,0.,0.));
#31346=CARTESIAN_POINT('',(1.8,0.,90.92));
#31347=CARTESIAN_POINT('',(1.8,0.,0.));
#31348=CARTESIAN_POINT('',(1.8,15.,90.92));
#31349=CARTESIAN_POINT('Origin',(1.8,0.,0.));
#31350=CARTESIAN_POINT('',(1.8,60.,90.92));
#31351=CARTESIAN_POINT('',(1.8,15.,90.92));
#31352=CARTESIAN_POINT('',(1.8,60.,0.));
#31353=CARTESIAN_POINT('Origin',(1.555,30.,90.92));
#31354=CARTESIAN_POINT('',(0.7775,0.,90.92));
#31355=CARTESIAN_POINT('Origin',(1.555,30.,90.92));
#31356=CARTESIAN_POINT('',(1.6775,60.,90.92));
#31357=CARTESIAN_POINT('Origin',(1.555,30.,89.08));
#31358=CARTESIAN_POINT('',(1.8,0.,89.08));
#31359=CARTESIAN_POINT('',(0.7775,0.,89.08));
#31360=CARTESIAN_POINT('',(1.8,15.,89.08));
#31361=CARTESIAN_POINT('Origin',(1.555,30.,89.08));
#31362=CARTESIAN_POINT('',(1.8,60.,89.08));
#31363=CARTESIAN_POINT('',(1.8,15.,89.08));
#31364=CARTESIAN_POINT('',(1.6775,60.,89.08));
#31365=CARTESIAN_POINT('Origin',(1.8,0.,0.));
#31366=CARTESIAN_POINT('',(1.8,0.,45.92));
#31367=CARTESIAN_POINT('',(1.8,0.,0.));
#31368=CARTESIAN_POINT('',(1.8,15.,45.92));
#31369=CARTESIAN_POINT('Origin',(1.8,0.,0.));
#31370=CARTESIAN_POINT('',(1.8,60.,45.92));
#31371=CARTESIAN_POINT('',(1.8,15.,45.92));
#31372=CARTESIAN_POINT('',(1.8,60.,0.));
#31373=CARTESIAN_POINT('Origin',(1.555,30.,45.92));
#31374=CARTESIAN_POINT('',(0.7775,0.,45.92));
#31375=CARTESIAN_POINT('Origin',(1.555,30.,45.92));
#31376=CARTESIAN_POINT('',(1.6775,60.,45.92));
#31377=CARTESIAN_POINT('Origin',(1.555,30.,44.08));
#31378=CARTESIAN_POINT('',(1.8,0.,44.08));
#31379=CARTESIAN_POINT('',(0.7775,0.,44.08));
#31380=CARTESIAN_POINT('',(1.8,15.,44.08));
#31381=CARTESIAN_POINT('Origin',(1.555,30.,44.08));
#31382=CARTESIAN_POINT('',(1.8,60.,44.08));
#31383=CARTESIAN_POINT('',(1.8,15.,44.08));
#31384=CARTESIAN_POINT('',(1.6775,60.,44.08));
#31385=CARTESIAN_POINT('Origin',(1.8,0.,0.));
#31386=CARTESIAN_POINT('',(1.8,0.,1.82));
#31387=CARTESIAN_POINT('',(1.8,0.,0.));
#31388=CARTESIAN_POINT('',(1.8,15.,1.82));
#31389=CARTESIAN_POINT('Origin',(1.8,0.,0.));
#31390=CARTESIAN_POINT('',(1.8,60.,1.82));
#31391=CARTESIAN_POINT('',(1.8,15.,1.82));
#31392=CARTESIAN_POINT('',(1.8,60.,0.));
#31393=CARTESIAN_POINT('Origin',(1.555,30.,1.82));
#31394=CARTESIAN_POINT('',(0.7775,0.,1.82));
#31395=CARTESIAN_POINT('Origin',(1.555,30.,1.82));
#31396=CARTESIAN_POINT('',(1.6775,60.,1.82));
#31397=CARTESIAN_POINT('Origin',(1.8,60.,0.));
#31398=CARTESIAN_POINT('',(0.,60.,0.));
#31399=CARTESIAN_POINT('',(1.8,60.,0.));
#31400=CARTESIAN_POINT('',(0.,60.,180.));
#31401=CARTESIAN_POINT('',(0.,60.,0.));
#31402=CARTESIAN_POINT('',(1.8,60.,180.));
#31403=CARTESIAN_POINT('Origin',(0.9,30.,0.));
#31404=CARTESIAN_POINT('',(0.,0.,0.));
#31405=CARTESIAN_POINT('',(0.,0.,0.));
#31406=CARTESIAN_POINT('',(0.,60.,0.));
#31407=CARTESIAN_POINT('Origin',(0.,0.,0.));
#31408=CARTESIAN_POINT('',(0.,0.,180.));
#31409=CARTESIAN_POINT('',(0.,0.,180.));
#31410=CARTESIAN_POINT('',(0.,0.,0.));
#31411=CARTESIAN_POINT('Origin',(0.,60.,0.));
#31412=CARTESIAN_POINT('',(0.,60.,180.));
#31413=CARTESIAN_POINT('Origin',(0.9,30.,180.));
#31545=UNCERTAINTY_MEASURE_WITH_UNIT(LENGTH_MEASURE(0.001),#31567,
'DISTANCE_ACCURACY_VALUE',
'Maximum model space distance between geometric entities at asserted c
onnectivities');
#31549=UNCERTAINTY_MEASURE_WITH_UNIT(LENGTH_MEASURE(0.001),#31567,
'DISTANCE_ACCURACY_VALUE',
'Maximum model space distance between geometric entities at asserted c
onnectivities');
#31562=(
GEOMETRIC_REPRESENTATION_CONTEXT(3)
GLOBAL_UNCERTAINTY_ASSIGNED_CONTEXT((#31545))
GLOBAL_UNIT_ASSIGNED_CONTEXT((#31567,#31569,#31570))
REPRESENTATION_CONTEXT('','3D')
);
#31566=(
GEOMETRIC_REPRESENTATION_CONTEXT(3)
GLOBAL_UNCERTAINTY_ASSIGNED_CONTEXT((#31549))
GLOBAL_UNIT_ASSIGNED_CONTEXT((#31567,#31569,#31570))
REPRESENTATION_CONTEXT('','3D')
);
#31567=(
LENGTH_UNIT()
NAMED_UNIT(*)
SI_UNIT(.CENTI.,.METRE.)
);
#31569=(
NAMED_UNIT(*)
PLANE_ANGLE_UNIT()
SI_UNIT($,.RADIAN.)
);
#31570=(
NAMED_UNIT(*)
SI_UNIT($,.STERADIAN.)
SOLID_ANGLE_UNIT()
);
#31583=SHAPE_DEFINITION_REPRESENTATION(#31599,#31647);
#31599=PRODUCT_DEFINITION_SHAPE('',$,#31664);
#31647=SHAPE_REPRESENTATION('',(#6171),#31562);
#31651=PRODUCT_DEFINITION_CONTEXT('part definition',#31701,'design');
#31664=PRODUCT_DEFINITION('Universal side panel_1',
'Universal side panel_Left',#31680,#31651);
#31680=PRODUCT_DEFINITION_FORMATION('',$,#31715);
#31701=APPLICATION_CONTEXT(
'Core Data for Automotive Mechanical Design Process');
#31702=PRODUCT_CONTEXT('part definition',#31701,'mechanical');
#31715=PRODUCT('Universal side panel_1','Universal side panel_Left',$,(#31702));
#31723=PRESENTATION_STYLE_ASSIGNMENT((#31730));
#31730=SURFACE_STYLE_USAGE(.BOTH.,#31737);
#31737=SURFACE_SIDE_STYLE('',(#31744));
#31744=SURFACE_STYLE_FILL_AREA(#31751);
#31751=FILL_AREA_STYLE('Opaque(24,59,110)',(#31758));
#31758=FILL_AREA_STYLE_COLOUR('Opaque(24,59,110)',#31765);
#31765=COLOUR_RGB('Opaque(24,59,110)',0.0941176470588235,0.231372549019608,
0.431372549019608);
ENDSEC;
END-ISO-10303-21;
